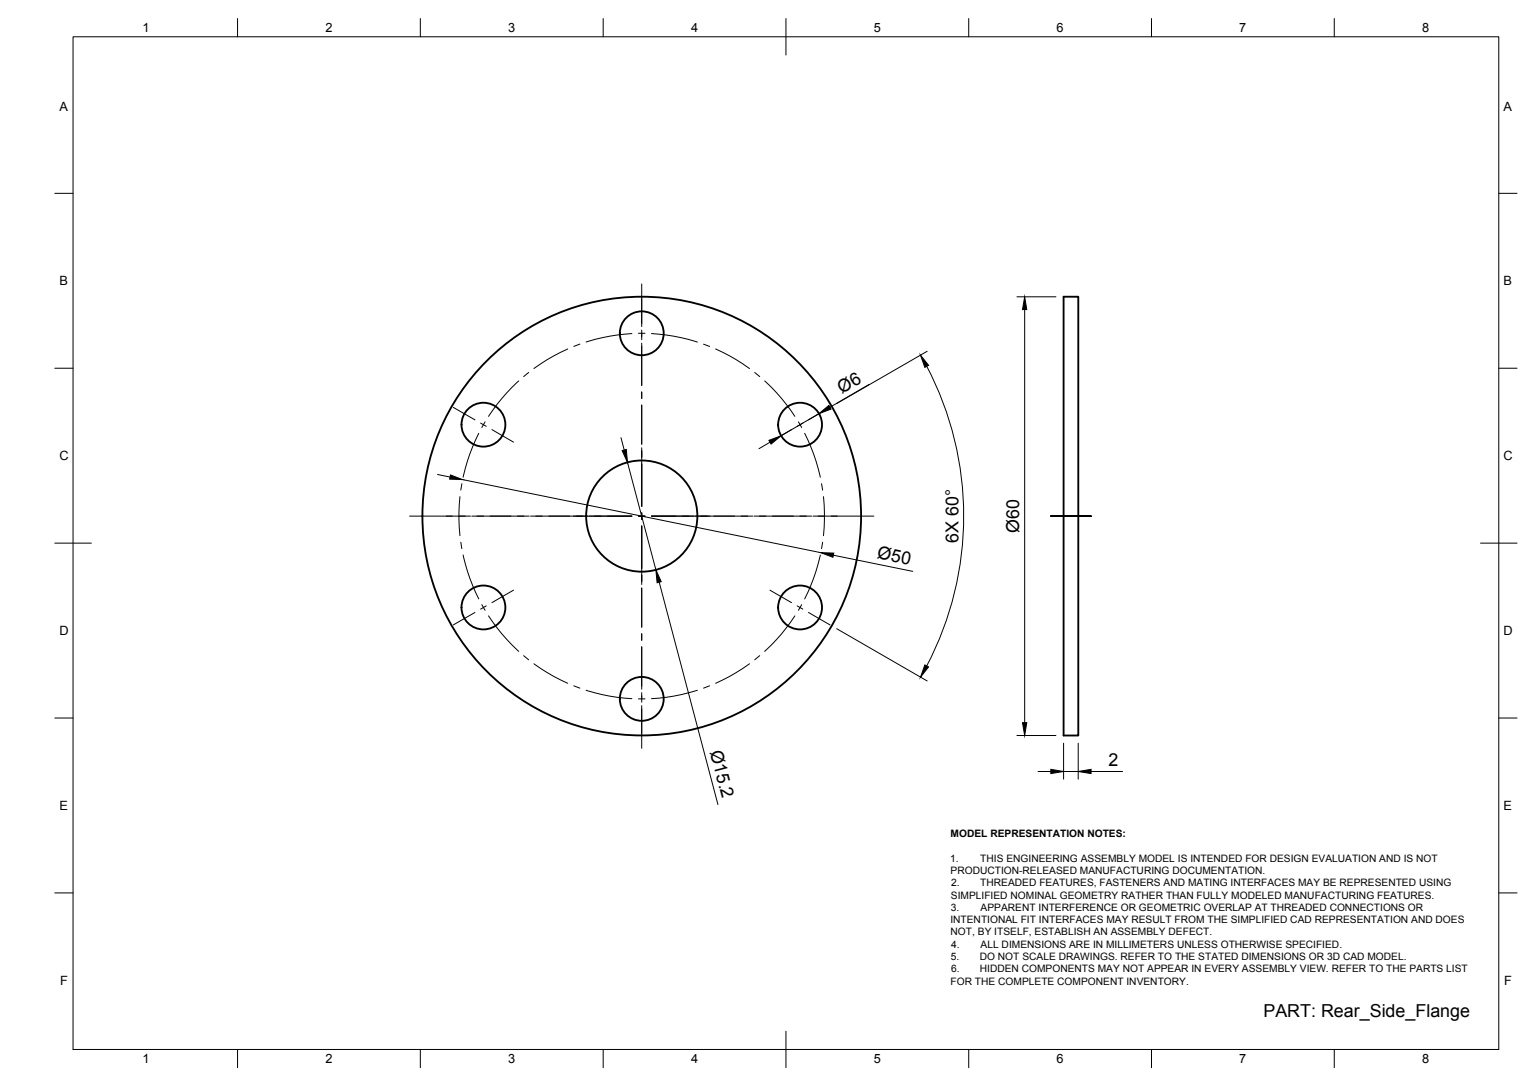
ISO-10303-21;
HEADER;
/* Generated by software containing ST-Developer
 * from STEP Tools, Inc. (www.steptools.com) 
 */

FILE_DESCRIPTION(
/* description */ ('STEP AP214'),
/* implementation_level */ '2;1');

FILE_NAME(
/* name */ 'Rear_Side_Flange.step',
/* time_stamp */ '2026-10-05T13:15:56-07:00',
/* author */ (''),
/* organization */ (''),
/* preprocessor_version */ 'ST-DEVELOPER v20.2',
/* originating_system */ 'Autodesk Translation Framework v15.15.0.0',
/* authorisation */ '');

FILE_SCHEMA (('AUTOMOTIVE_DESIGN { 1 0 10303 214 3 1 1 }'));
ENDSEC;

DATA;
#10=MECHANICAL_DESIGN_GEOMETRIC_PRESENTATION_REPRESENTATION('',(#1351),#37881);
#1327=SHAPE_REPRESENTATION_RELATIONSHIP('SRR','None',#37960,#1339);
#1339=ADVANCED_BREP_SHAPE_REPRESENTATION('',(#1363),#37875);
#1351=STYLED_ITEM('',(#38023),#1363);
#1363=MANIFOLD_SOLID_BREP('Body1',#10825);
#1433=FACE_BOUND('',#2791,.T.);
#1434=FACE_BOUND('',#2792,.T.);
#1435=FACE_BOUND('',#2793,.T.);
#1436=FACE_BOUND('',#2794,.T.);
#1437=FACE_BOUND('',#2795,.T.);
#1438=FACE_BOUND('',#2796,.T.);
#1439=FACE_BOUND('',#2797,.T.);
#1440=FACE_BOUND('',#2799,.T.);
#1441=FACE_BOUND('',#2800,.T.);
#1442=FACE_BOUND('',#2801,.T.);
#1443=FACE_BOUND('',#2802,.T.);
#1444=FACE_BOUND('',#2803,.T.);
#1445=FACE_BOUND('',#2804,.T.);
#1446=FACE_BOUND('',#2805,.T.);
#1531=PLANE('',#11765);
#1532=PLANE('',#11766);
#2117=FACE_OUTER_BOUND('',#2782,.T.);
#2118=FACE_OUTER_BOUND('',#2783,.T.);
#2119=FACE_OUTER_BOUND('',#2784,.T.);
#2120=FACE_OUTER_BOUND('',#2785,.T.);
#2121=FACE_OUTER_BOUND('',#2786,.T.);
#2122=FACE_OUTER_BOUND('',#2787,.T.);
#2123=FACE_OUTER_BOUND('',#2788,.T.);
#2124=FACE_OUTER_BOUND('',#2789,.T.);
#2125=FACE_OUTER_BOUND('',#2790,.T.);
#2126=FACE_OUTER_BOUND('',#2798,.T.);
#2782=EDGE_LOOP('',(#9773,#9774,#9775,#9776));
#2783=EDGE_LOOP('',(#9777,#9778,#9779,#9780));
#2784=EDGE_LOOP('',(#9781,#9782,#9783,#9784));
#2785=EDGE_LOOP('',(#9785,#9786,#9787,#9788));
#2786=EDGE_LOOP('',(#9789,#9790,#9791,#9792));
#2787=EDGE_LOOP('',(#9793,#9794,#9795,#9796));
#2788=EDGE_LOOP('',(#9797,#9798,#9799,#9800));
#2789=EDGE_LOOP('',(#9801,#9802,#9803,#9804));
#2790=EDGE_LOOP('',(#9805));
#2791=EDGE_LOOP('',(#9806));
#2792=EDGE_LOOP('',(#9807));
#2793=EDGE_LOOP('',(#9808));
#2794=EDGE_LOOP('',(#9809));
#2795=EDGE_LOOP('',(#9810));
#2796=EDGE_LOOP('',(#9811));
#2797=EDGE_LOOP('',(#9812));
#2798=EDGE_LOOP('',(#9813));
#2799=EDGE_LOOP('',(#9814));
#2800=EDGE_LOOP('',(#9815));
#2801=EDGE_LOOP('',(#9816));
#2802=EDGE_LOOP('',(#9817));
#2803=EDGE_LOOP('',(#9818));
#2804=EDGE_LOOP('',(#9819));
#2805=EDGE_LOOP('',(#9820));
#3090=LINE('',#37542,#3391);
#3091=LINE('',#37548,#3392);
#3092=LINE('',#37554,#3393);
#3093=LINE('',#37560,#3394);
#3094=LINE('',#37566,#3395);
#3095=LINE('',#37572,#3396);
#3096=LINE('',#37578,#3397);
#3097=LINE('',#37584,#3398);
#3391=VECTOR('',#13667,3.);
#3392=VECTOR('',#13674,3.);
#3393=VECTOR('',#13681,3.);
#3394=VECTOR('',#13688,3.00000000000001);
#3395=VECTOR('',#13695,3.);
#3396=VECTOR('',#13702,3.);
#3397=VECTOR('',#13709,7.6);
#3398=VECTOR('',#13716,30.);
#3952=CIRCLE('',#11742,3.);
#3953=CIRCLE('',#11743,3.);
#3954=CIRCLE('',#11745,3.);
#3955=CIRCLE('',#11746,3.);
#3956=CIRCLE('',#11748,3.);
#3957=CIRCLE('',#11749,3.);
#3958=CIRCLE('',#11751,3.00000000000001);
#3959=CIRCLE('',#11752,3.00000000000001);
#3960=CIRCLE('',#11754,3.);
#3961=CIRCLE('',#11755,3.);
#3962=CIRCLE('',#11757,3.);
#3963=CIRCLE('',#11758,3.);
#3964=CIRCLE('',#11760,7.6);
#3965=CIRCLE('',#11761,7.6);
#3966=CIRCLE('',#11763,30.);
#3967=CIRCLE('',#11764,30.);
#4988=VERTEX_POINT('',#37539);
#4989=VERTEX_POINT('',#37541);
#4990=VERTEX_POINT('',#37545);
#4991=VERTEX_POINT('',#37547);
#4992=VERTEX_POINT('',#37551);
#4993=VERTEX_POINT('',#37553);
#4994=VERTEX_POINT('',#37557);
#4995=VERTEX_POINT('',#37559);
#4996=VERTEX_POINT('',#37563);
#4997=VERTEX_POINT('',#37565);
#4998=VERTEX_POINT('',#37569);
#4999=VERTEX_POINT('',#37571);
#5000=VERTEX_POINT('',#37575);
#5001=VERTEX_POINT('',#37577);
#5002=VERTEX_POINT('',#37581);
#5003=VERTEX_POINT('',#37583);
#6597=EDGE_CURVE('',#4988,#4988,#3952,.T.);
#6598=EDGE_CURVE('',#4988,#4989,#3090,.T.);
#6599=EDGE_CURVE('',#4989,#4989,#3953,.T.);
#6600=EDGE_CURVE('',#4990,#4990,#3954,.T.);
#6601=EDGE_CURVE('',#4990,#4991,#3091,.T.);
#6602=EDGE_CURVE('',#4991,#4991,#3955,.T.);
#6603=EDGE_CURVE('',#4992,#4992,#3956,.T.);
#6604=EDGE_CURVE('',#4992,#4993,#3092,.T.);
#6605=EDGE_CURVE('',#4993,#4993,#3957,.T.);
#6606=EDGE_CURVE('',#4994,#4994,#3958,.T.);
#6607=EDGE_CURVE('',#4994,#4995,#3093,.T.);
#6608=EDGE_CURVE('',#4995,#4995,#3959,.T.);
#6609=EDGE_CURVE('',#4996,#4996,#3960,.T.);
#6610=EDGE_CURVE('',#4996,#4997,#3094,.T.);
#6611=EDGE_CURVE('',#4997,#4997,#3961,.T.);
#6612=EDGE_CURVE('',#4998,#4998,#3962,.T.);
#6613=EDGE_CURVE('',#4998,#4999,#3095,.T.);
#6614=EDGE_CURVE('',#4999,#4999,#3963,.T.);
#6615=EDGE_CURVE('',#5000,#5000,#3964,.T.);
#6616=EDGE_CURVE('',#5000,#5001,#3096,.T.);
#6617=EDGE_CURVE('',#5001,#5001,#3965,.T.);
#6618=EDGE_CURVE('',#5002,#5002,#3966,.T.);
#6619=EDGE_CURVE('',#5002,#5003,#3097,.T.);
#6620=EDGE_CURVE('',#5003,#5003,#3967,.T.);
#9773=ORIENTED_EDGE('',*,*,#6597,.T.);
#9774=ORIENTED_EDGE('',*,*,#6598,.T.);
#9775=ORIENTED_EDGE('',*,*,#6599,.F.);
#9776=ORIENTED_EDGE('',*,*,#6598,.F.);
#9777=ORIENTED_EDGE('',*,*,#6600,.T.);
#9778=ORIENTED_EDGE('',*,*,#6601,.T.);
#9779=ORIENTED_EDGE('',*,*,#6602,.F.);
#9780=ORIENTED_EDGE('',*,*,#6601,.F.);
#9781=ORIENTED_EDGE('',*,*,#6603,.T.);
#9782=ORIENTED_EDGE('',*,*,#6604,.T.);
#9783=ORIENTED_EDGE('',*,*,#6605,.F.);
#9784=ORIENTED_EDGE('',*,*,#6604,.F.);
#9785=ORIENTED_EDGE('',*,*,#6606,.T.);
#9786=ORIENTED_EDGE('',*,*,#6607,.T.);
#9787=ORIENTED_EDGE('',*,*,#6608,.F.);
#9788=ORIENTED_EDGE('',*,*,#6607,.F.);
#9789=ORIENTED_EDGE('',*,*,#6609,.T.);
#9790=ORIENTED_EDGE('',*,*,#6610,.T.);
#9791=ORIENTED_EDGE('',*,*,#6611,.F.);
#9792=ORIENTED_EDGE('',*,*,#6610,.F.);
#9793=ORIENTED_EDGE('',*,*,#6612,.T.);
#9794=ORIENTED_EDGE('',*,*,#6613,.T.);
#9795=ORIENTED_EDGE('',*,*,#6614,.F.);
#9796=ORIENTED_EDGE('',*,*,#6613,.F.);
#9797=ORIENTED_EDGE('',*,*,#6615,.T.);
#9798=ORIENTED_EDGE('',*,*,#6616,.T.);
#9799=ORIENTED_EDGE('',*,*,#6617,.F.);
#9800=ORIENTED_EDGE('',*,*,#6616,.F.);
#9801=ORIENTED_EDGE('',*,*,#6618,.T.);
#9802=ORIENTED_EDGE('',*,*,#6619,.T.);
#9803=ORIENTED_EDGE('',*,*,#6620,.F.);
#9804=ORIENTED_EDGE('',*,*,#6619,.F.);
#9805=ORIENTED_EDGE('',*,*,#6620,.T.);
#9806=ORIENTED_EDGE('',*,*,#6615,.F.);
#9807=ORIENTED_EDGE('',*,*,#6609,.F.);
#9808=ORIENTED_EDGE('',*,*,#6603,.F.);
#9809=ORIENTED_EDGE('',*,*,#6597,.F.);
#9810=ORIENTED_EDGE('',*,*,#6600,.F.);
#9811=ORIENTED_EDGE('',*,*,#6606,.F.);
#9812=ORIENTED_EDGE('',*,*,#6612,.F.);
#9813=ORIENTED_EDGE('',*,*,#6618,.F.);
#9814=ORIENTED_EDGE('',*,*,#6617,.T.);
#9815=ORIENTED_EDGE('',*,*,#6614,.T.);
#9816=ORIENTED_EDGE('',*,*,#6611,.T.);
#9817=ORIENTED_EDGE('',*,*,#6608,.T.);
#9818=ORIENTED_EDGE('',*,*,#6605,.T.);
#9819=ORIENTED_EDGE('',*,*,#6602,.T.);
#9820=ORIENTED_EDGE('',*,*,#6599,.T.);
#10189=CYLINDRICAL_SURFACE('',#11741,3.);
#10190=CYLINDRICAL_SURFACE('',#11744,3.);
#10191=CYLINDRICAL_SURFACE('',#11747,3.);
#10192=CYLINDRICAL_SURFACE('',#11750,3.00000000000001);
#10193=CYLINDRICAL_SURFACE('',#11753,3.);
#10194=CYLINDRICAL_SURFACE('',#11756,3.);
#10195=CYLINDRICAL_SURFACE('',#11759,7.6);
#10196=CYLINDRICAL_SURFACE('',#11762,30.);
#10762=ADVANCED_FACE('',(#2117),#10189,.F.);
#10763=ADVANCED_FACE('',(#2118),#10190,.F.);
#10764=ADVANCED_FACE('',(#2119),#10191,.F.);
#10765=ADVANCED_FACE('',(#2120),#10192,.F.);
#10766=ADVANCED_FACE('',(#2121),#10193,.F.);
#10767=ADVANCED_FACE('',(#2122),#10194,.F.);
#10768=ADVANCED_FACE('',(#2123),#10195,.F.);
#10769=ADVANCED_FACE('',(#2124),#10196,.T.);
#10770=ADVANCED_FACE('',(#2125,#1433,#1434,#1435,#1436,#1437,#1438,#1439),
#1531,.T.);
#10771=ADVANCED_FACE('',(#2126,#1440,#1441,#1442,#1443,#1444,#1445,#1446),
#1532,.F.);
#10825=CLOSED_SHELL('',(#10762,#10763,#10764,#10765,#10766,#10767,#10768,
#10769,#10770,#10771));
#11740=AXIS2_PLACEMENT_3D('',#37537,#13661,#13662);
#11741=AXIS2_PLACEMENT_3D('',#37538,#13663,#13664);
#11742=AXIS2_PLACEMENT_3D('',#37540,#13665,#13666);
#11743=AXIS2_PLACEMENT_3D('',#37543,#13668,#13669);
#11744=AXIS2_PLACEMENT_3D('',#37544,#13670,#13671);
#11745=AXIS2_PLACEMENT_3D('',#37546,#13672,#13673);
#11746=AXIS2_PLACEMENT_3D('',#37549,#13675,#13676);
#11747=AXIS2_PLACEMENT_3D('',#37550,#13677,#13678);
#11748=AXIS2_PLACEMENT_3D('',#37552,#13679,#13680);
#11749=AXIS2_PLACEMENT_3D('',#37555,#13682,#13683);
#11750=AXIS2_PLACEMENT_3D('',#37556,#13684,#13685);
#11751=AXIS2_PLACEMENT_3D('',#37558,#13686,#13687);
#11752=AXIS2_PLACEMENT_3D('',#37561,#13689,#13690);
#11753=AXIS2_PLACEMENT_3D('',#37562,#13691,#13692);
#11754=AXIS2_PLACEMENT_3D('',#37564,#13693,#13694);
#11755=AXIS2_PLACEMENT_3D('',#37567,#13696,#13697);
#11756=AXIS2_PLACEMENT_3D('',#37568,#13698,#13699);
#11757=AXIS2_PLACEMENT_3D('',#37570,#13700,#13701);
#11758=AXIS2_PLACEMENT_3D('',#37573,#13703,#13704);
#11759=AXIS2_PLACEMENT_3D('',#37574,#13705,#13706);
#11760=AXIS2_PLACEMENT_3D('',#37576,#13707,#13708);
#11761=AXIS2_PLACEMENT_3D('',#37579,#13710,#13711);
#11762=AXIS2_PLACEMENT_3D('',#37580,#13712,#13713);
#11763=AXIS2_PLACEMENT_3D('',#37582,#13714,#13715);
#11764=AXIS2_PLACEMENT_3D('',#37585,#13717,#13718);
#11765=AXIS2_PLACEMENT_3D('',#37586,#13719,#13720);
#11766=AXIS2_PLACEMENT_3D('',#37587,#13721,#13722);
#13661=DIRECTION('axis',(0.,0.,1.));
#13662=DIRECTION('refdir',(1.,0.,0.));
#13663=DIRECTION('center_axis',(0.,0.,-1.));
#13664=DIRECTION('ref_axis',(-1.,0.,0.));
#13665=DIRECTION('center_axis',(0.,0.,1.));
#13666=DIRECTION('ref_axis',(1.,0.,0.));
#13667=DIRECTION('',(0.,0.,-1.));
#13668=DIRECTION('center_axis',(0.,0.,1.));
#13669=DIRECTION('ref_axis',(1.,0.,0.));
#13670=DIRECTION('center_axis',(0.,0.,-1.));
#13671=DIRECTION('ref_axis',(-1.,0.,0.));
#13672=DIRECTION('center_axis',(0.,0.,1.));
#13673=DIRECTION('ref_axis',(1.,0.,0.));
#13674=DIRECTION('',(0.,0.,-1.));
#13675=DIRECTION('center_axis',(0.,0.,1.));
#13676=DIRECTION('ref_axis',(1.,0.,0.));
#13677=DIRECTION('center_axis',(0.,0.,-1.));
#13678=DIRECTION('ref_axis',(-1.,0.,0.));
#13679=DIRECTION('center_axis',(0.,0.,1.));
#13680=DIRECTION('ref_axis',(1.,0.,0.));
#13681=DIRECTION('',(0.,0.,-1.));
#13682=DIRECTION('center_axis',(0.,0.,1.));
#13683=DIRECTION('ref_axis',(1.,0.,0.));
#13684=DIRECTION('center_axis',(0.,0.,-1.));
#13685=DIRECTION('ref_axis',(-1.,0.,0.));
#13686=DIRECTION('center_axis',(0.,0.,1.));
#13687=DIRECTION('ref_axis',(1.,0.,0.));
#13688=DIRECTION('',(0.,0.,-1.));
#13689=DIRECTION('center_axis',(0.,0.,1.));
#13690=DIRECTION('ref_axis',(1.,0.,0.));
#13691=DIRECTION('center_axis',(0.,0.,-1.));
#13692=DIRECTION('ref_axis',(-1.,0.,0.));
#13693=DIRECTION('center_axis',(0.,0.,1.));
#13694=DIRECTION('ref_axis',(1.,0.,0.));
#13695=DIRECTION('',(0.,0.,-1.));
#13696=DIRECTION('center_axis',(0.,0.,1.));
#13697=DIRECTION('ref_axis',(1.,0.,0.));
#13698=DIRECTION('center_axis',(0.,0.,-1.));
#13699=DIRECTION('ref_axis',(-1.,0.,0.));
#13700=DIRECTION('center_axis',(0.,0.,1.));
#13701=DIRECTION('ref_axis',(1.,0.,0.));
#13702=DIRECTION('',(0.,0.,-1.));
#13703=DIRECTION('center_axis',(0.,0.,1.));
#13704=DIRECTION('ref_axis',(1.,0.,0.));
#13705=DIRECTION('center_axis',(0.,0.,-1.));
#13706=DIRECTION('ref_axis',(-1.,0.,0.));
#13707=DIRECTION('center_axis',(0.,0.,1.));
#13708=DIRECTION('ref_axis',(1.,0.,0.));
#13709=DIRECTION('',(0.,0.,-1.));
#13710=DIRECTION('center_axis',(0.,0.,1.));
#13711=DIRECTION('ref_axis',(1.,0.,0.));
#13712=DIRECTION('center_axis',(0.,0.,-1.));
#13713=DIRECTION('ref_axis',(-1.,0.,0.));
#13714=DIRECTION('center_axis',(0.,0.,1.));
#13715=DIRECTION('ref_axis',(1.,0.,0.));
#13716=DIRECTION('',(0.,0.,1.));
#13717=DIRECTION('center_axis',(0.,0.,1.));
#13718=DIRECTION('ref_axis',(1.,0.,0.));
#13719=DIRECTION('center_axis',(0.,0.,1.));
#13720=DIRECTION('ref_axis',(1.,0.,0.));
#13721=DIRECTION('center_axis',(0.,0.,1.));
#13722=DIRECTION('ref_axis',(1.,0.,0.));
#37537=CARTESIAN_POINT('',(0.,0.,0.));
#37538=CARTESIAN_POINT('Origin',(-21.650635094611,12.5,1.));
#37539=CARTESIAN_POINT('',(-18.650635094611,12.5,1.));
#37540=CARTESIAN_POINT('Origin',(-21.650635094611,12.5,1.));
#37541=CARTESIAN_POINT('',(-18.650635094611,12.5,-1.));
#37542=CARTESIAN_POINT('',(-18.650635094611,12.5,1.));
#37543=CARTESIAN_POINT('Origin',(-21.650635094611,12.5,-1.));
#37544=CARTESIAN_POINT('Origin',(-21.650635094611,-12.5,1.));
#37545=CARTESIAN_POINT('',(-18.650635094611,-12.5,1.));
#37546=CARTESIAN_POINT('Origin',(-21.650635094611,-12.5,1.));
#37547=CARTESIAN_POINT('',(-18.650635094611,-12.5,-1.));
#37548=CARTESIAN_POINT('',(-18.650635094611,-12.5,1.));
#37549=CARTESIAN_POINT('Origin',(-21.650635094611,-12.5,-1.));
#37550=CARTESIAN_POINT('Origin',(3.46944695195361E-15,-25.,1.));
#37551=CARTESIAN_POINT('',(3.,-25.,1.));
#37552=CARTESIAN_POINT('Origin',(3.46944695195361E-15,-25.,1.));
#37553=CARTESIAN_POINT('',(3.,-25.,-1.));
#37554=CARTESIAN_POINT('',(3.,-25.,1.));
#37555=CARTESIAN_POINT('Origin',(3.46944695195361E-15,-25.,-1.));
#37556=CARTESIAN_POINT('Origin',(21.650635094611,-12.5,1.));
#37557=CARTESIAN_POINT('',(24.650635094611,-12.5,1.));
#37558=CARTESIAN_POINT('Origin',(21.650635094611,-12.5,1.));
#37559=CARTESIAN_POINT('',(24.650635094611,-12.5,-1.));
#37560=CARTESIAN_POINT('',(24.650635094611,-12.5,1.));
#37561=CARTESIAN_POINT('Origin',(21.650635094611,-12.5,-1.));
#37562=CARTESIAN_POINT('Origin',(21.650635094611,12.5,1.));
#37563=CARTESIAN_POINT('',(24.650635094611,12.5,1.));
#37564=CARTESIAN_POINT('Origin',(21.650635094611,12.5,1.));
#37565=CARTESIAN_POINT('',(24.650635094611,12.5,-1.));
#37566=CARTESIAN_POINT('',(24.650635094611,12.5,1.));
#37567=CARTESIAN_POINT('Origin',(21.650635094611,12.5,-1.));
#37568=CARTESIAN_POINT('Origin',(0.,25.,1.));
#37569=CARTESIAN_POINT('',(3.,25.,1.));
#37570=CARTESIAN_POINT('Origin',(0.,25.,1.));
#37571=CARTESIAN_POINT('',(3.,25.,-1.));
#37572=CARTESIAN_POINT('',(3.,25.,1.));
#37573=CARTESIAN_POINT('Origin',(0.,25.,-1.));
#37574=CARTESIAN_POINT('Origin',(0.,0.,1.));
#37575=CARTESIAN_POINT('',(7.6,-9.30731567351989E-16,1.));
#37576=CARTESIAN_POINT('Origin',(0.,0.,1.));
#37577=CARTESIAN_POINT('',(7.6,-9.30731567351989E-16,-1.));
#37578=CARTESIAN_POINT('',(7.6,-9.30731567351989E-16,1.));
#37579=CARTESIAN_POINT('Origin',(0.,0.,-1.));
#37580=CARTESIAN_POINT('Origin',(0.,0.,1.));
#37581=CARTESIAN_POINT('',(30.,-3.67394039744206E-15,-1.));
#37582=CARTESIAN_POINT('Origin',(0.,0.,-1.));
#37583=CARTESIAN_POINT('',(30.,-3.67394039744206E-15,1.));
#37584=CARTESIAN_POINT('',(30.,-3.67394039744206E-15,1.));
#37585=CARTESIAN_POINT('Origin',(0.,0.,1.));
#37586=CARTESIAN_POINT('Origin',(0.,0.,1.));
#37587=CARTESIAN_POINT('Origin',(0.,0.,-1.));
#37861=UNCERTAINTY_MEASURE_WITH_UNIT(LENGTH_MEASURE(0.01),#37882,
'DISTANCE_ACCURACY_VALUE',
'Maximum model space distance between geometric entities at asserted c
onnectivities');
#37867=UNCERTAINTY_MEASURE_WITH_UNIT(LENGTH_MEASURE(0.01),#37882,
'DISTANCE_ACCURACY_VALUE',
'Maximum model space distance between geometric entities at asserted c
onnectivities');
#37875=(
GEOMETRIC_REPRESENTATION_CONTEXT(3)
GLOBAL_UNCERTAINTY_ASSIGNED_CONTEXT((#37861))
GLOBAL_UNIT_ASSIGNED_CONTEXT((#37882,#37884,#37885))
REPRESENTATION_CONTEXT('','3D')
);
#37881=(
GEOMETRIC_REPRESENTATION_CONTEXT(3)
GLOBAL_UNCERTAINTY_ASSIGNED_CONTEXT((#37867))
GLOBAL_UNIT_ASSIGNED_CONTEXT((#37882,#37884,#37885))
REPRESENTATION_CONTEXT('','3D')
);
#37882=(
LENGTH_UNIT()
NAMED_UNIT(*)
SI_UNIT(.MILLI.,.METRE.)
);
#37884=(
NAMED_UNIT(*)
PLANE_ANGLE_UNIT()
SI_UNIT($,.RADIAN.)
);
#37885=(
NAMED_UNIT(*)
SI_UNIT($,.STERADIAN.)
SOLID_ANGLE_UNIT()
);
#37893=SHAPE_DEFINITION_REPRESENTATION(#37906,#37960);
#37906=PRODUCT_DEFINITION_SHAPE('',$,#37974);
#37960=SHAPE_REPRESENTATION('',(#11740),#37875);
#37966=PRODUCT_DEFINITION_CONTEXT('part definition',#38007,'design');
#37974=PRODUCT_DEFINITION('PS10','Rear_Side_Flange',#37987,#37966);
#37987=PRODUCT_DEFINITION_FORMATION('',$,#38016);
#38007=APPLICATION_CONTEXT(
'Core Data for Automotive Mechanical Design Process');
#38008=PRODUCT_CONTEXT('part definition',#38007,'mechanical');
#38016=PRODUCT('PS10','Rear_Side_Flange',$,(#38008));
#38023=PRESENTATION_STYLE_ASSIGNMENT((#38025));
#38025=SURFACE_STYLE_USAGE(.BOTH.,#38027);
#38027=SURFACE_SIDE_STYLE('',(#38029));
#38029=SURFACE_STYLE_FILL_AREA(#38031);
#38031=FILL_AREA_STYLE('Opaque(202,209,238)',(#38033));
#38033=FILL_AREA_STYLE_COLOUR('Opaque(202,209,238)',#38035);
#38035=COLOUR_RGB('Opaque(202,209,238)', 0.66274510, 0.83137255, 0.94901961);
ENDSEC;
END-ISO-10303-21;
